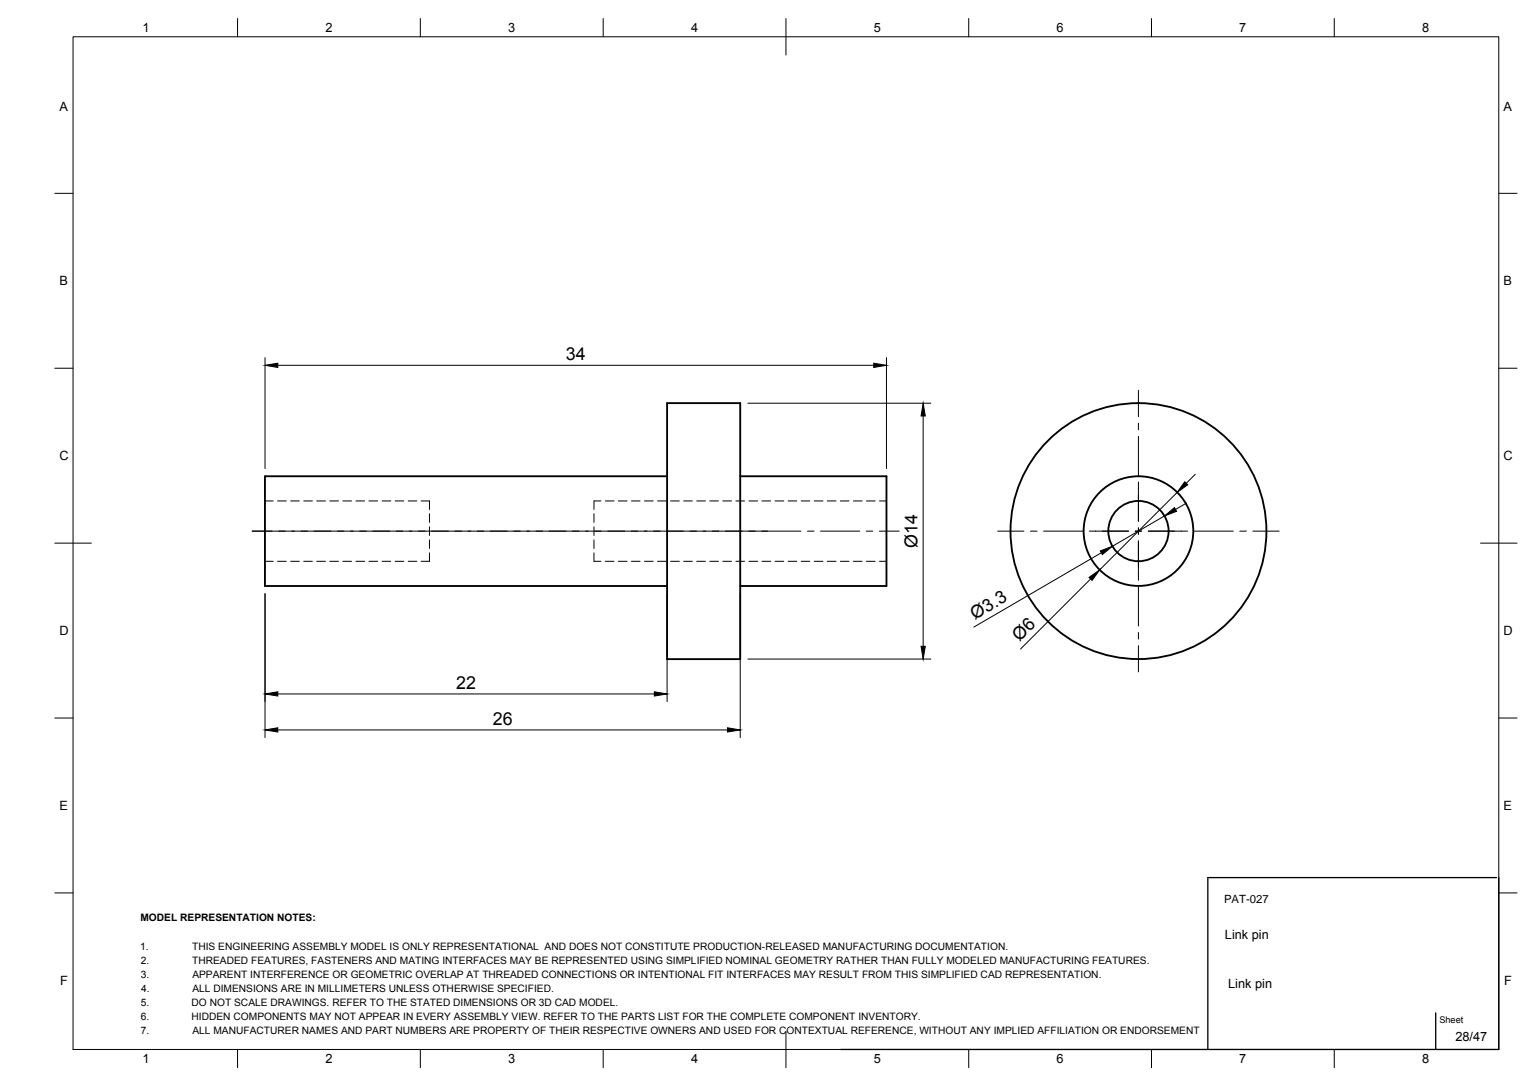
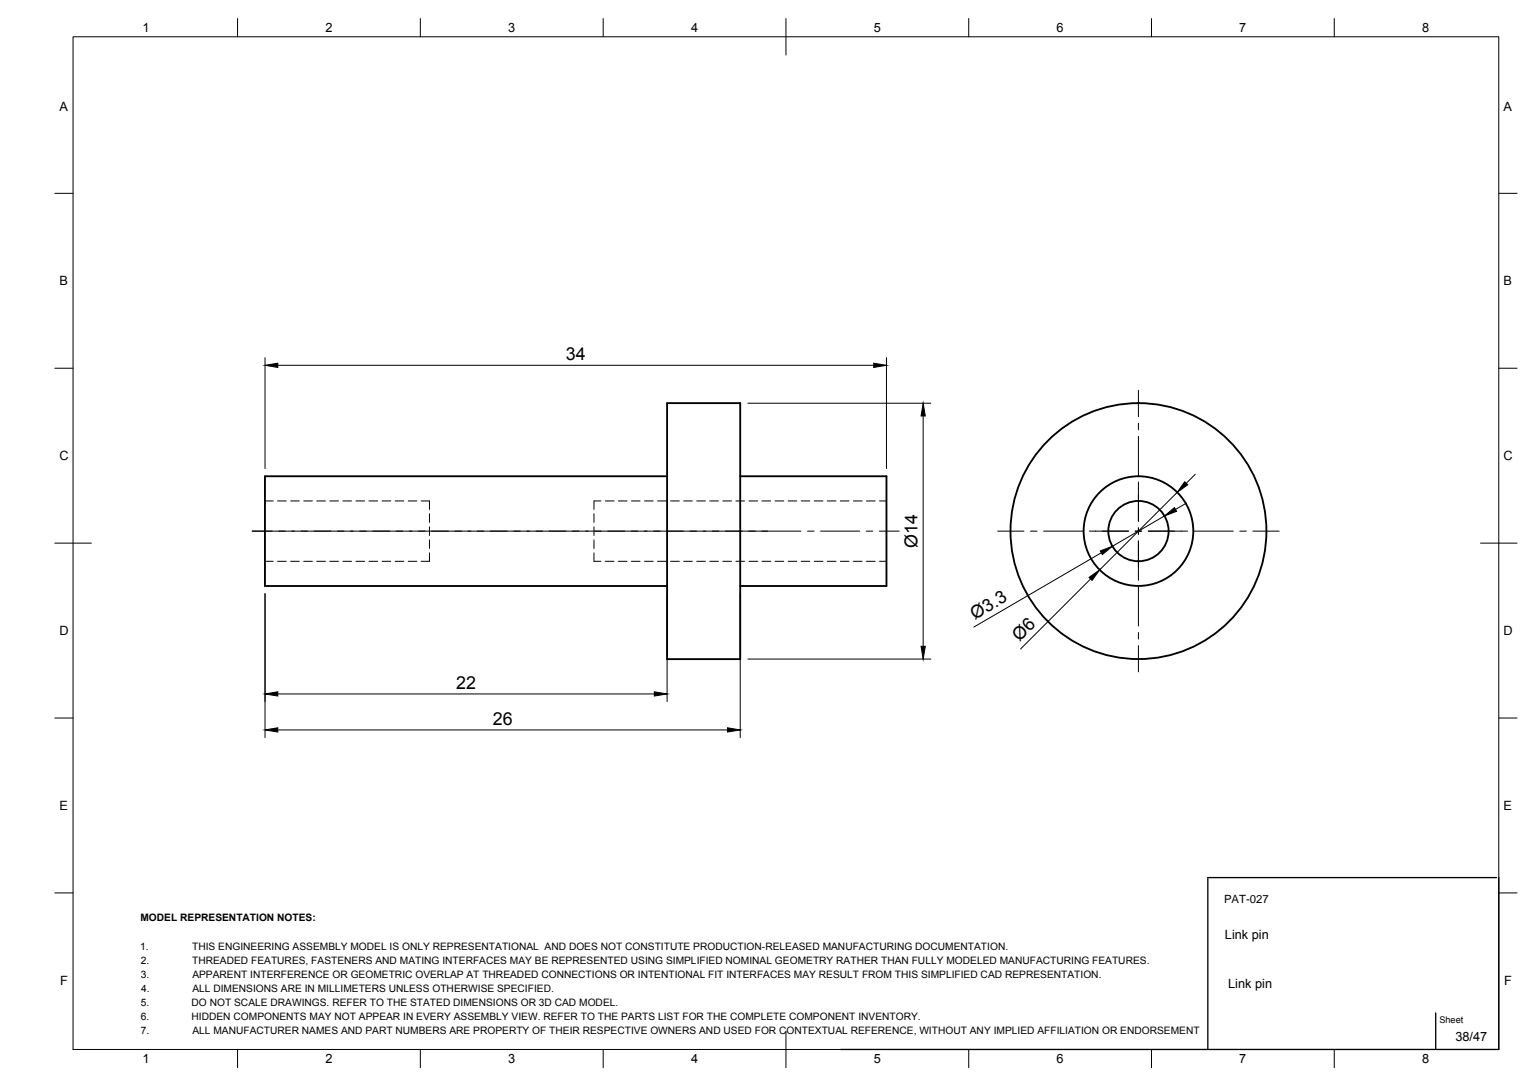
ISO-10303-21;
HEADER;
/* Generated by software containing ST-Developer
 * from STEP Tools, Inc. (www.steptools.com) 
 */

FILE_DESCRIPTION(
/* description */ ('Crank-driven oscillating fan base (mechanism only)'),

/* implementation_level */ '2;1');

FILE_NAME(
/* name */ 'Link pin.step',
/* time_stamp */ '2026-10-28T03:25:00-07:00',
/* author */ (''),
/* organization */ (''),
/* preprocessor_version */ 'ST-DEVELOPER v20.2',
/* originating_system */ 'Autodesk Translation Framework v15.17.0.0',
/* authorisation */ '');

FILE_SCHEMA (('AUTOMOTIVE_DESIGN { 1 0 10303 214 3 1 1 }'));
ENDSEC;

DATA;
#10=MECHANICAL_DESIGN_GEOMETRIC_PRESENTATION_REPRESENTATION('',(#465),#11916);
#377=SHAPE_REPRESENTATION_RELATIONSHIP('SRR','None',#12103,#417);
#417=ADVANCED_BREP_SHAPE_REPRESENTATION('',(#512),#11894);
#465=STYLED_ITEM('',(#12375),#512);
#512=MANIFOLD_SOLID_BREP('Body1',#6096);
#636=FACE_BOUND('',#1588,.T.);
#637=FACE_BOUND('',#1590,.T.);
#638=FACE_BOUND('',#1595,.T.);
#639=FACE_BOUND('',#1597,.T.);
#792=PLANE('',#7053);
#793=PLANE('',#7057);
#794=PLANE('',#7058);
#795=PLANE('',#7061);
#796=PLANE('',#7069);
#797=PLANE('',#7070);
#1102=FACE_OUTER_BOUND('',#1583,.T.);
#1103=FACE_OUTER_BOUND('',#1584,.T.);
#1104=FACE_OUTER_BOUND('',#1585,.T.);
#1105=FACE_OUTER_BOUND('',#1586,.T.);
#1106=FACE_OUTER_BOUND('',#1587,.T.);
#1107=FACE_OUTER_BOUND('',#1589,.T.);
#1108=FACE_OUTER_BOUND('',#1591,.T.);
#1109=FACE_OUTER_BOUND('',#1592,.T.);
#1110=FACE_OUTER_BOUND('',#1593,.T.);
#1111=FACE_OUTER_BOUND('',#1594,.T.);
#1112=FACE_OUTER_BOUND('',#1596,.T.);
#1583=EDGE_LOOP('',(#4970,#4971,#4972,#4973));
#1584=EDGE_LOOP('',(#4974));
#1585=EDGE_LOOP('',(#4975,#4976,#4977,#4978));
#1586=EDGE_LOOP('',(#4979));
#1587=EDGE_LOOP('',(#4980));
#1588=EDGE_LOOP('',(#4981));
#1589=EDGE_LOOP('',(#4982));
#1590=EDGE_LOOP('',(#4983));
#1591=EDGE_LOOP('',(#4984,#4985,#4986,#4987));
#1592=EDGE_LOOP('',(#4988,#4989,#4990,#4991));
#1593=EDGE_LOOP('',(#4992,#4993,#4994,#4995));
#1594=EDGE_LOOP('',(#4996));
#1595=EDGE_LOOP('',(#4997));
#1596=EDGE_LOOP('',(#4998));
#1597=EDGE_LOOP('',(#4999));
#1968=LINE('',#11048,#2301);
#1969=LINE('',#11055,#2302);
#1970=LINE('',#11069,#2303);
#1971=LINE('',#11072,#2304);
#1972=LINE('',#11077,#2305);
#2301=VECTOR('',#8567,0.165);
#2302=VECTOR('',#8576,0.165);
#2303=VECTOR('',#8595,0.7);
#2304=VECTOR('',#8598,0.3);
#2305=VECTOR('',#8605,0.3);
#2709=CIRCLE('',#7051,0.165);
#2710=CIRCLE('',#7052,0.165);
#2711=CIRCLE('',#7055,0.165);
#2712=CIRCLE('',#7056,0.165);
#2713=CIRCLE('',#7059,0.7);
#2714=CIRCLE('',#7060,0.3);
#2715=CIRCLE('',#7062,0.7);
#2716=CIRCLE('',#7063,0.3);
#2717=CIRCLE('',#7066,0.3);
#2718=CIRCLE('',#7068,0.3);
#3140=VERTEX_POINT('',#11045);
#3141=VERTEX_POINT('',#11047);
#3142=VERTEX_POINT('',#11052);
#3143=VERTEX_POINT('',#11054);
#3144=VERTEX_POINT('',#11059);
#3145=VERTEX_POINT('',#11061);
#3146=VERTEX_POINT('',#11064);
#3147=VERTEX_POINT('',#11066);
#3148=VERTEX_POINT('',#11071);
#3149=VERTEX_POINT('',#11075);
#3780=EDGE_CURVE('',#3140,#3140,#2709,.T.);
#3781=EDGE_CURVE('',#3140,#3141,#1968,.T.);
#3782=EDGE_CURVE('',#3141,#3141,#2710,.T.);
#3783=EDGE_CURVE('',#3142,#3142,#2711,.T.);
#3784=EDGE_CURVE('',#3142,#3143,#1969,.T.);
#3785=EDGE_CURVE('',#3143,#3143,#2712,.T.);
#3786=EDGE_CURVE('',#3144,#3144,#2713,.T.);
#3787=EDGE_CURVE('',#3145,#3145,#2714,.T.);
#3788=EDGE_CURVE('',#3146,#3146,#2715,.T.);
#3789=EDGE_CURVE('',#3147,#3147,#2716,.T.);
#3790=EDGE_CURVE('',#3144,#3146,#1970,.T.);
#3791=EDGE_CURVE('',#3147,#3148,#1971,.T.);
#3792=EDGE_CURVE('',#3148,#3148,#2717,.T.);
#3793=EDGE_CURVE('',#3149,#3149,#2718,.T.);
#3794=EDGE_CURVE('',#3149,#3145,#1972,.T.);
#4970=ORIENTED_EDGE('',*,*,#3780,.F.);
#4971=ORIENTED_EDGE('',*,*,#3781,.T.);
#4972=ORIENTED_EDGE('',*,*,#3782,.F.);
#4973=ORIENTED_EDGE('',*,*,#3781,.F.);
#4974=ORIENTED_EDGE('',*,*,#3780,.T.);
#4975=ORIENTED_EDGE('',*,*,#3783,.F.);
#4976=ORIENTED_EDGE('',*,*,#3784,.T.);
#4977=ORIENTED_EDGE('',*,*,#3785,.T.);
#4978=ORIENTED_EDGE('',*,*,#3784,.F.);
#4979=ORIENTED_EDGE('',*,*,#3785,.F.);
#4980=ORIENTED_EDGE('',*,*,#3786,.T.);
#4981=ORIENTED_EDGE('',*,*,#3787,.F.);
#4982=ORIENTED_EDGE('',*,*,#3788,.F.);
#4983=ORIENTED_EDGE('',*,*,#3789,.F.);
#4984=ORIENTED_EDGE('',*,*,#3786,.F.);
#4985=ORIENTED_EDGE('',*,*,#3790,.T.);
#4986=ORIENTED_EDGE('',*,*,#3788,.T.);
#4987=ORIENTED_EDGE('',*,*,#3790,.F.);
#4988=ORIENTED_EDGE('',*,*,#3789,.T.);
#4989=ORIENTED_EDGE('',*,*,#3791,.T.);
#4990=ORIENTED_EDGE('',*,*,#3792,.T.);
#4991=ORIENTED_EDGE('',*,*,#3791,.F.);
#4992=ORIENTED_EDGE('',*,*,#3793,.F.);
#4993=ORIENTED_EDGE('',*,*,#3794,.T.);
#4994=ORIENTED_EDGE('',*,*,#3787,.T.);
#4995=ORIENTED_EDGE('',*,*,#3794,.F.);
#4996=ORIENTED_EDGE('',*,*,#3793,.T.);
#4997=ORIENTED_EDGE('',*,*,#3782,.T.);
#4998=ORIENTED_EDGE('',*,*,#3792,.F.);
#4999=ORIENTED_EDGE('',*,*,#3783,.T.);
#5637=CYLINDRICAL_SURFACE('',#7050,0.165);
#5638=CYLINDRICAL_SURFACE('',#7054,0.165);
#5639=CYLINDRICAL_SURFACE('',#7064,0.7);
#5640=CYLINDRICAL_SURFACE('',#7065,0.3);
#5641=CYLINDRICAL_SURFACE('',#7067,0.3);
#5908=ADVANCED_FACE('',(#1102),#5637,.F.);
#5909=ADVANCED_FACE('',(#1103),#792,.T.);
#5910=ADVANCED_FACE('',(#1104),#5638,.F.);
#5911=ADVANCED_FACE('',(#1105),#793,.F.);
#5912=ADVANCED_FACE('',(#1106,#636),#794,.T.);
#5913=ADVANCED_FACE('',(#1107,#637),#795,.F.);
#5914=ADVANCED_FACE('',(#1108),#5639,.T.);
#5915=ADVANCED_FACE('',(#1109),#5640,.T.);
#5916=ADVANCED_FACE('',(#1110),#5641,.T.);
#5917=ADVANCED_FACE('',(#1111,#638),#796,.T.);
#5918=ADVANCED_FACE('',(#1112,#639),#797,.F.);
#6096=CLOSED_SHELL('',(#5908,#5909,#5910,#5911,#5912,#5913,#5914,#5915,
#5916,#5917,#5918));
#7049=AXIS2_PLACEMENT_3D('',#11043,#8561,#8562);
#7050=AXIS2_PLACEMENT_3D('',#11044,#8563,#8564);
#7051=AXIS2_PLACEMENT_3D('',#11046,#8565,#8566);
#7052=AXIS2_PLACEMENT_3D('',#11049,#8568,#8569);
#7053=AXIS2_PLACEMENT_3D('',#11050,#8570,#8571);
#7054=AXIS2_PLACEMENT_3D('',#11051,#8572,#8573);
#7055=AXIS2_PLACEMENT_3D('',#11053,#8574,#8575);
#7056=AXIS2_PLACEMENT_3D('',#11056,#8577,#8578);
#7057=AXIS2_PLACEMENT_3D('',#11057,#8579,#8580);
#7058=AXIS2_PLACEMENT_3D('',#11058,#8581,#8582);
#7059=AXIS2_PLACEMENT_3D('',#11060,#8583,#8584);
#7060=AXIS2_PLACEMENT_3D('',#11062,#8585,#8586);
#7061=AXIS2_PLACEMENT_3D('',#11063,#8587,#8588);
#7062=AXIS2_PLACEMENT_3D('',#11065,#8589,#8590);
#7063=AXIS2_PLACEMENT_3D('',#11067,#8591,#8592);
#7064=AXIS2_PLACEMENT_3D('',#11068,#8593,#8594);
#7065=AXIS2_PLACEMENT_3D('',#11070,#8596,#8597);
#7066=AXIS2_PLACEMENT_3D('',#11073,#8599,#8600);
#7067=AXIS2_PLACEMENT_3D('',#11074,#8601,#8602);
#7068=AXIS2_PLACEMENT_3D('',#11076,#8603,#8604);
#7069=AXIS2_PLACEMENT_3D('',#11078,#8606,#8607);
#7070=AXIS2_PLACEMENT_3D('',#11079,#8608,#8609);
#8561=DIRECTION('axis',(0.,0.,1.));
#8562=DIRECTION('refdir',(1.,0.,0.));
#8563=DIRECTION('center_axis',(0.,0.,1.));
#8564=DIRECTION('ref_axis',(1.,0.,0.));
#8565=DIRECTION('center_axis',(0.,0.,1.));
#8566=DIRECTION('ref_axis',(1.,0.,0.));
#8567=DIRECTION('',(0.,0.,1.));
#8568=DIRECTION('center_axis',(0.,0.,-1.));
#8569=DIRECTION('ref_axis',(1.,0.,0.));
#8570=DIRECTION('center_axis',(0.,0.,1.));
#8571=DIRECTION('ref_axis',(1.,0.,0.));
#8572=DIRECTION('center_axis',(0.,0.,1.));
#8573=DIRECTION('ref_axis',(1.,0.,0.));
#8574=DIRECTION('center_axis',(0.,0.,1.));
#8575=DIRECTION('ref_axis',(1.,0.,0.));
#8576=DIRECTION('',(0.,0.,1.));
#8577=DIRECTION('center_axis',(0.,0.,1.));
#8578=DIRECTION('ref_axis',(1.,0.,0.));
#8579=DIRECTION('center_axis',(0.,0.,1.));
#8580=DIRECTION('ref_axis',(1.,0.,0.));
#8581=DIRECTION('center_axis',(0.,0.,1.));
#8582=DIRECTION('ref_axis',(1.,0.,0.));
#8583=DIRECTION('center_axis',(0.,0.,1.));
#8584=DIRECTION('ref_axis',(1.,0.,0.));
#8585=DIRECTION('center_axis',(0.,0.,1.));
#8586=DIRECTION('ref_axis',(1.,0.,0.));
#8587=DIRECTION('center_axis',(0.,0.,1.));
#8588=DIRECTION('ref_axis',(1.,0.,0.));
#8589=DIRECTION('center_axis',(0.,0.,1.));
#8590=DIRECTION('ref_axis',(1.,0.,0.));
#8591=DIRECTION('center_axis',(0.,0.,-1.));
#8592=DIRECTION('ref_axis',(1.,0.,0.));
#8593=DIRECTION('center_axis',(0.,0.,1.));
#8594=DIRECTION('ref_axis',(1.,0.,0.));
#8595=DIRECTION('',(0.,0.,-1.));
#8596=DIRECTION('center_axis',(0.,0.,1.));
#8597=DIRECTION('ref_axis',(1.,0.,0.));
#8598=DIRECTION('',(0.,0.,-1.));
#8599=DIRECTION('center_axis',(0.,0.,1.));
#8600=DIRECTION('ref_axis',(1.,0.,0.));
#8601=DIRECTION('center_axis',(0.,0.,1.));
#8602=DIRECTION('ref_axis',(1.,0.,0.));
#8603=DIRECTION('center_axis',(0.,0.,1.));
#8604=DIRECTION('ref_axis',(1.,0.,0.));
#8605=DIRECTION('',(0.,0.,-1.));
#8606=DIRECTION('center_axis',(0.,0.,1.));
#8607=DIRECTION('ref_axis',(1.,0.,0.));
#8608=DIRECTION('center_axis',(0.,0.,1.));
#8609=DIRECTION('ref_axis',(1.,0.,0.));
#11043=CARTESIAN_POINT('',(0.,0.,0.));
#11044=CARTESIAN_POINT('Origin',(-0.429855350392604,2.61349944954989,8.7));
#11045=CARTESIAN_POINT('',(-0.594855350392604,2.61349944954989,8.7));
#11046=CARTESIAN_POINT('Origin',(-0.429855350392604,2.61349944954989,8.7));
#11047=CARTESIAN_POINT('',(-0.594855350392604,2.61349944954989,9.6));
#11048=CARTESIAN_POINT('',(-0.594855350392604,2.61349944954989,8.7));
#11049=CARTESIAN_POINT('Origin',(-0.429855350392604,2.61349944954989,9.6));
#11050=CARTESIAN_POINT('Origin',(-0.429855350392604,2.61349944954989,8.7));
#11051=CARTESIAN_POINT('Origin',(-0.429855350392604,2.61349944954989,6.1));
#11052=CARTESIAN_POINT('',(-0.594855350392604,2.61349944954989,6.2));
#11053=CARTESIAN_POINT('Origin',(-0.429855350392604,2.61349944954989,6.2));
#11054=CARTESIAN_POINT('',(-0.594855350392604,2.61349944954989,7.8));
#11055=CARTESIAN_POINT('',(-0.594855350392604,2.61349944954989,6.1));
#11056=CARTESIAN_POINT('Origin',(-0.429855350392604,2.61349944954989,7.8));
#11057=CARTESIAN_POINT('Origin',(-0.429855350392604,2.61349944954989,7.8));
#11058=CARTESIAN_POINT('Origin',(-0.429855350392604,2.61349944954989,7.4));
#11059=CARTESIAN_POINT('',(-1.1298553503926,2.61349944954989,7.4));
#11060=CARTESIAN_POINT('Origin',(-0.429855350392604,2.61349944954989,7.4));
#11061=CARTESIAN_POINT('',(-0.729855350392604,2.61349944954989,7.4));
#11062=CARTESIAN_POINT('Origin',(-0.429855350392604,2.61349944954989,7.4));
#11063=CARTESIAN_POINT('Origin',(-0.429855350392604,2.61349944954989,7.));
#11064=CARTESIAN_POINT('',(-1.1298553503926,2.61349944954989,7.));
#11065=CARTESIAN_POINT('Origin',(-0.429855350392604,2.61349944954989,7.));
#11066=CARTESIAN_POINT('',(-0.729855350392604,2.61349944954989,7.));
#11067=CARTESIAN_POINT('Origin',(-0.429855350392604,2.61349944954989,7.));
#11068=CARTESIAN_POINT('Origin',(-0.429855350392604,2.61349944954989,7.));
#11069=CARTESIAN_POINT('',(-1.1298553503926,2.61349944954989,7.));
#11070=CARTESIAN_POINT('Origin',(-0.429855350392604,2.61349944954989,6.2));
#11071=CARTESIAN_POINT('',(-0.729855350392604,2.61349944954989,6.2));
#11072=CARTESIAN_POINT('',(-0.729855350392604,2.61349944954989,6.2));
#11073=CARTESIAN_POINT('Origin',(-0.429855350392604,2.61349944954989,6.2));
#11074=CARTESIAN_POINT('Origin',(-0.429855350392604,2.61349944954989,6.2));
#11075=CARTESIAN_POINT('',(-0.729855350392604,2.61349944954989,9.6));
#11076=CARTESIAN_POINT('Origin',(-0.429855350392604,2.61349944954989,9.6));
#11077=CARTESIAN_POINT('',(-0.729855350392604,2.61349944954989,6.2));
#11078=CARTESIAN_POINT('Origin',(-0.429855350392604,2.61349944954989,9.6));
#11079=CARTESIAN_POINT('Origin',(-0.429855350392604,2.61349944954989,6.2));
#11847=UNCERTAINTY_MEASURE_WITH_UNIT(LENGTH_MEASURE(0.001),#11917,
'DISTANCE_ACCURACY_VALUE',
'Maximum model space distance between geometric entities at asserted c
onnectivities');
#11869=UNCERTAINTY_MEASURE_WITH_UNIT(LENGTH_MEASURE(0.001),#11917,
'DISTANCE_ACCURACY_VALUE',
'Maximum model space distance between geometric entities at asserted c
onnectivities');
#11894=(
GEOMETRIC_REPRESENTATION_CONTEXT(3)
GLOBAL_UNCERTAINTY_ASSIGNED_CONTEXT((#11847))
GLOBAL_UNIT_ASSIGNED_CONTEXT((#11917,#11919,#11920))
REPRESENTATION_CONTEXT('','3D')
);
#11916=(
GEOMETRIC_REPRESENTATION_CONTEXT(3)
GLOBAL_UNCERTAINTY_ASSIGNED_CONTEXT((#11869))
GLOBAL_UNIT_ASSIGNED_CONTEXT((#11917,#11919,#11920))
REPRESENTATION_CONTEXT('','3D')
);
#11917=(
LENGTH_UNIT()
NAMED_UNIT(*)
SI_UNIT(.CENTI.,.METRE.)
);
#11919=(
NAMED_UNIT(*)
PLANE_ANGLE_UNIT()
SI_UNIT($,.RADIAN.)
);
#11920=(
NAMED_UNIT(*)
SI_UNIT($,.STERADIAN.)
SOLID_ANGLE_UNIT()
);
#11945=SHAPE_DEFINITION_REPRESENTATION(#11996,#12103);
#11996=PRODUCT_DEFINITION_SHAPE('',$,#12150);
#12103=SHAPE_REPRESENTATION('',(#7049),#11894);
#12125=PRODUCT_DEFINITION_CONTEXT('part definition',#12265,'design');
#12150=PRODUCT_DEFINITION('Link pin','Link pin',#12196,#12125);
#12196=PRODUCT_DEFINITION_FORMATION('',$,#12291);
#12265=APPLICATION_CONTEXT(
'Core Data for Automotive Mechanical Design Process');
#12266=PRODUCT_CONTEXT('part definition',#12265,'mechanical');
#12291=PRODUCT('Link pin','Link pin','Link pin',(#12266));
#12369=COLOUR_RGB('Grey',0.48,0.52,0.57);
#12370=FILL_AREA_STYLE_COLOUR('',#12369);
#12371=FILL_AREA_STYLE('',(#12370));
#12372=SURFACE_STYLE_FILL_AREA(#12371);
#12373=SURFACE_SIDE_STYLE('',(#12372));
#12374=SURFACE_STYLE_USAGE(.BOTH.,#12373);
#12375=PRESENTATION_STYLE_ASSIGNMENT((#12374));
ENDSEC;
END-ISO-10303-21;
